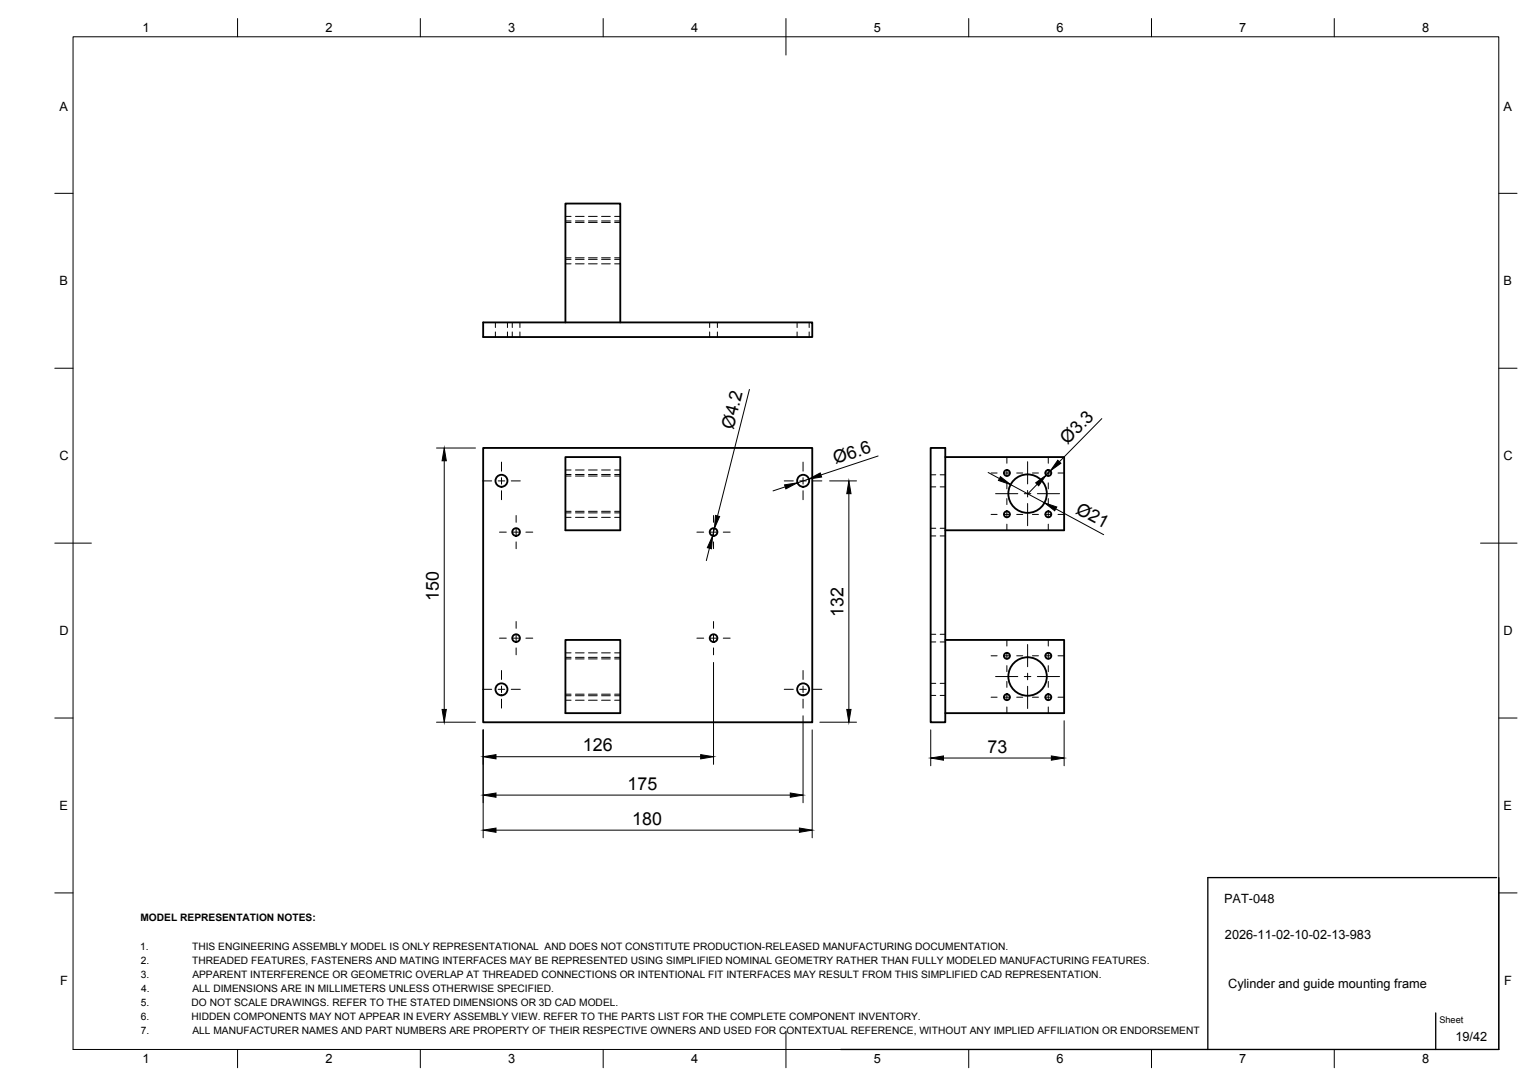
ISO-10303-21;
HEADER;
/* Generated by software containing ST-Developer
 * from STEP Tools, Inc. (www.steptools.com) 
 */

FILE_DESCRIPTION(
/* description */ ('Guided pneumatic stop gate'),
/* implementation_level */ '2;1');

FILE_NAME(
/* name */ 'Cylinder and guide mounting frame.step',
/* time_stamp */ '2026-10-27T21:43:45-07:00',
/* author */ (''),
/* organization */ (''),
/* preprocessor_version */ 'ST-DEVELOPER v20.2',
/* originating_system */ 'Autodesk Translation Framework v15.17.0.0',
/* authorisation */ '');

FILE_SCHEMA (('AUTOMOTIVE_DESIGN { 1 0 10303 214 3 1 1 }'));
ENDSEC;

DATA;
#10=MECHANICAL_DESIGN_GEOMETRIC_PRESENTATION_REPRESENTATION('',(#554),#14392);
#470=SHAPE_REPRESENTATION_RELATIONSHIP('SRR','None',#14605,#512);
#512=ADVANCED_BREP_SHAPE_REPRESENTATION('',(#595),#14367);
#554=STYLED_ITEM('',(#14870),#595);
#595=MANIFOLD_SOLID_BREP('Body1',#7895);
#699=FACE_BOUND('',#1926,.T.);
#700=FACE_BOUND('',#1927,.T.);
#701=FACE_BOUND('',#1928,.T.);
#702=FACE_BOUND('',#1929,.T.);
#703=FACE_BOUND('',#1930,.T.);
#704=FACE_BOUND('',#1932,.T.);
#705=FACE_BOUND('',#1933,.T.);
#706=FACE_BOUND('',#1934,.T.);
#707=FACE_BOUND('',#1935,.T.);
#708=FACE_BOUND('',#1936,.T.);
#709=FACE_BOUND('',#1946,.T.);
#710=FACE_BOUND('',#1947,.T.);
#711=FACE_BOUND('',#1948,.T.);
#712=FACE_BOUND('',#1949,.T.);
#713=FACE_BOUND('',#1950,.T.);
#714=FACE_BOUND('',#1952,.T.);
#715=FACE_BOUND('',#1953,.T.);
#716=FACE_BOUND('',#1954,.T.);
#717=FACE_BOUND('',#1955,.T.);
#718=FACE_BOUND('',#1956,.T.);
#719=FACE_BOUND('',#1962,.T.);
#720=FACE_BOUND('',#1963,.T.);
#721=FACE_BOUND('',#1964,.T.);
#722=FACE_BOUND('',#1965,.T.);
#723=FACE_BOUND('',#1966,.T.);
#724=FACE_BOUND('',#1967,.T.);
#725=FACE_BOUND('',#1968,.T.);
#726=FACE_BOUND('',#1969,.T.);
#727=FACE_BOUND('',#1970,.T.);
#728=FACE_BOUND('',#1971,.T.);
#729=FACE_BOUND('',#1973,.T.);
#730=FACE_BOUND('',#1974,.T.);
#731=FACE_BOUND('',#1975,.T.);
#732=FACE_BOUND('',#1976,.T.);
#733=FACE_BOUND('',#1977,.T.);
#734=FACE_BOUND('',#1978,.T.);
#735=FACE_BOUND('',#1979,.T.);
#736=FACE_BOUND('',#1980,.T.);
#979=PLANE('',#8865);
#980=PLANE('',#8866);
#981=PLANE('',#8867);
#982=PLANE('',#8868);
#983=PLANE('',#8869);
#984=PLANE('',#8885);
#985=PLANE('',#8886);
#986=PLANE('',#8887);
#987=PLANE('',#8888);
#988=PLANE('',#8889);
#989=PLANE('',#8890);
#990=PLANE('',#8891);
#991=PLANE('',#8892);
#992=PLANE('',#8893);
#993=PLANE('',#8894);
#994=PLANE('',#8895);
#1350=FACE_OUTER_BOUND('',#1909,.T.);
#1351=FACE_OUTER_BOUND('',#1910,.T.);
#1352=FACE_OUTER_BOUND('',#1911,.T.);
#1353=FACE_OUTER_BOUND('',#1912,.T.);
#1354=FACE_OUTER_BOUND('',#1913,.T.);
#1355=FACE_OUTER_BOUND('',#1914,.T.);
#1356=FACE_OUTER_BOUND('',#1915,.T.);
#1357=FACE_OUTER_BOUND('',#1916,.T.);
#1358=FACE_OUTER_BOUND('',#1917,.T.);
#1359=FACE_OUTER_BOUND('',#1918,.T.);
#1360=FACE_OUTER_BOUND('',#1919,.T.);
#1361=FACE_OUTER_BOUND('',#1920,.T.);
#1362=FACE_OUTER_BOUND('',#1921,.T.);
#1363=FACE_OUTER_BOUND('',#1922,.T.);
#1364=FACE_OUTER_BOUND('',#1923,.T.);
#1365=FACE_OUTER_BOUND('',#1924,.T.);
#1366=FACE_OUTER_BOUND('',#1925,.T.);
#1367=FACE_OUTER_BOUND('',#1931,.T.);
#1368=FACE_OUTER_BOUND('',#1937,.T.);
#1369=FACE_OUTER_BOUND('',#1938,.T.);
#1370=FACE_OUTER_BOUND('',#1939,.T.);
#1371=FACE_OUTER_BOUND('',#1940,.T.);
#1372=FACE_OUTER_BOUND('',#1941,.T.);
#1373=FACE_OUTER_BOUND('',#1942,.T.);
#1374=FACE_OUTER_BOUND('',#1943,.T.);
#1375=FACE_OUTER_BOUND('',#1944,.T.);
#1376=FACE_OUTER_BOUND('',#1945,.T.);
#1377=FACE_OUTER_BOUND('',#1951,.T.);
#1378=FACE_OUTER_BOUND('',#1957,.T.);
#1379=FACE_OUTER_BOUND('',#1958,.T.);
#1380=FACE_OUTER_BOUND('',#1959,.T.);
#1381=FACE_OUTER_BOUND('',#1960,.T.);
#1382=FACE_OUTER_BOUND('',#1961,.T.);
#1383=FACE_OUTER_BOUND('',#1972,.T.);
#1909=EDGE_LOOP('',(#6222,#6223,#6224,#6225));
#1910=EDGE_LOOP('',(#6226,#6227,#6228,#6229));
#1911=EDGE_LOOP('',(#6230,#6231,#6232,#6233));
#1912=EDGE_LOOP('',(#6234,#6235,#6236,#6237));
#1913=EDGE_LOOP('',(#6238,#6239,#6240,#6241));
#1914=EDGE_LOOP('',(#6242,#6243,#6244,#6245));
#1915=EDGE_LOOP('',(#6246,#6247,#6248,#6249));
#1916=EDGE_LOOP('',(#6250,#6251,#6252,#6253));
#1917=EDGE_LOOP('',(#6254,#6255,#6256,#6257));
#1918=EDGE_LOOP('',(#6258,#6259,#6260,#6261));
#1919=EDGE_LOOP('',(#6262,#6263,#6264,#6265));
#1920=EDGE_LOOP('',(#6266,#6267,#6268,#6269));
#1921=EDGE_LOOP('',(#6270,#6271,#6272,#6273));
#1922=EDGE_LOOP('',(#6274,#6275,#6276,#6277));
#1923=EDGE_LOOP('',(#6278,#6279,#6280,#6281));
#1924=EDGE_LOOP('',(#6282,#6283,#6284,#6285));
#1925=EDGE_LOOP('',(#6286,#6287,#6288,#6289));
#1926=EDGE_LOOP('',(#6290));
#1927=EDGE_LOOP('',(#6291));
#1928=EDGE_LOOP('',(#6292));
#1929=EDGE_LOOP('',(#6293));
#1930=EDGE_LOOP('',(#6294));
#1931=EDGE_LOOP('',(#6295,#6296,#6297,#6298));
#1932=EDGE_LOOP('',(#6299));
#1933=EDGE_LOOP('',(#6300));
#1934=EDGE_LOOP('',(#6301));
#1935=EDGE_LOOP('',(#6302));
#1936=EDGE_LOOP('',(#6303));
#1937=EDGE_LOOP('',(#6304,#6305,#6306,#6307));
#1938=EDGE_LOOP('',(#6308,#6309,#6310,#6311));
#1939=EDGE_LOOP('',(#6312,#6313,#6314,#6315));
#1940=EDGE_LOOP('',(#6316,#6317,#6318,#6319));
#1941=EDGE_LOOP('',(#6320,#6321,#6322,#6323));
#1942=EDGE_LOOP('',(#6324,#6325,#6326,#6327));
#1943=EDGE_LOOP('',(#6328,#6329,#6330,#6331));
#1944=EDGE_LOOP('',(#6332,#6333,#6334,#6335));
#1945=EDGE_LOOP('',(#6336,#6337,#6338,#6339));
#1946=EDGE_LOOP('',(#6340));
#1947=EDGE_LOOP('',(#6341));
#1948=EDGE_LOOP('',(#6342));
#1949=EDGE_LOOP('',(#6343));
#1950=EDGE_LOOP('',(#6344));
#1951=EDGE_LOOP('',(#6345,#6346,#6347,#6348));
#1952=EDGE_LOOP('',(#6349));
#1953=EDGE_LOOP('',(#6350));
#1954=EDGE_LOOP('',(#6351));
#1955=EDGE_LOOP('',(#6352));
#1956=EDGE_LOOP('',(#6353));
#1957=EDGE_LOOP('',(#6354,#6355,#6356,#6357));
#1958=EDGE_LOOP('',(#6358,#6359,#6360,#6361));
#1959=EDGE_LOOP('',(#6362,#6363,#6364,#6365));
#1960=EDGE_LOOP('',(#6366,#6367,#6368,#6369));
#1961=EDGE_LOOP('',(#6370,#6371,#6372,#6373));
#1962=EDGE_LOOP('',(#6374,#6375,#6376,#6377));
#1963=EDGE_LOOP('',(#6378,#6379,#6380,#6381));
#1964=EDGE_LOOP('',(#6382));
#1965=EDGE_LOOP('',(#6383));
#1966=EDGE_LOOP('',(#6384));
#1967=EDGE_LOOP('',(#6385));
#1968=EDGE_LOOP('',(#6386));
#1969=EDGE_LOOP('',(#6387));
#1970=EDGE_LOOP('',(#6388));
#1971=EDGE_LOOP('',(#6389));
#1972=EDGE_LOOP('',(#6390,#6391,#6392,#6393));
#1973=EDGE_LOOP('',(#6394));
#1974=EDGE_LOOP('',(#6395));
#1975=EDGE_LOOP('',(#6396));
#1976=EDGE_LOOP('',(#6397));
#1977=EDGE_LOOP('',(#6398));
#1978=EDGE_LOOP('',(#6399));
#1979=EDGE_LOOP('',(#6400));
#1980=EDGE_LOOP('',(#6401));
#2534=LINE('',#12945,#3079);
#2535=LINE('',#12951,#3080);
#2536=LINE('',#12957,#3081);
#2537=LINE('',#12963,#3082);
#2538=LINE('',#12969,#3083);
#2539=LINE('',#12975,#3084);
#2540=LINE('',#12981,#3085);
#2541=LINE('',#12987,#3086);
#2542=LINE('',#12993,#3087);
#2543=LINE('',#12999,#3088);
#2544=LINE('',#13005,#3089);
#2545=LINE('',#13011,#3090);
#2546=LINE('',#13017,#3091);
#2547=LINE('',#13022,#3092);
#2548=LINE('',#13024,#3093);
#2549=LINE('',#13026,#3094);
#2550=LINE('',#13027,#3095);
#2551=LINE('',#13031,#3096);
#2552=LINE('',#13033,#3097);
#2553=LINE('',#13035,#3098);
#2554=LINE('',#13036,#3099);
#2555=LINE('',#13038,#3100);
#2556=LINE('',#13039,#3101);
#2557=LINE('',#13041,#3102);
#2558=LINE('',#13043,#3103);
#2559=LINE('',#13048,#3104);
#2560=LINE('',#13054,#3105);
#2561=LINE('',#13060,#3106);
#2562=LINE('',#13066,#3107);
#2563=LINE('',#13072,#3108);
#2564=LINE('',#13077,#3109);
#2565=LINE('',#13079,#3110);
#2566=LINE('',#13081,#3111);
#2567=LINE('',#13082,#3112);
#2568=LINE('',#13086,#3113);
#2569=LINE('',#13088,#3114);
#2570=LINE('',#13090,#3115);
#2571=LINE('',#13091,#3116);
#2572=LINE('',#13093,#3117);
#2573=LINE('',#13094,#3118);
#2574=LINE('',#13096,#3119);
#2575=LINE('',#13098,#3120);
#2576=LINE('',#13102,#3121);
#2577=LINE('',#13104,#3122);
#2578=LINE('',#13106,#3123);
#2579=LINE('',#13107,#3124);
#2580=LINE('',#13110,#3125);
#2581=LINE('',#13112,#3126);
#2582=LINE('',#13113,#3127);
#2583=LINE('',#13116,#3128);
#2584=LINE('',#13118,#3129);
#2585=LINE('',#13119,#3130);
#2586=LINE('',#13121,#3131);
#2587=LINE('',#13122,#3132);
#3079=VECTOR('',#10525,0.33);
#3080=VECTOR('',#10532,0.33);
#3081=VECTOR('',#10539,0.33);
#3082=VECTOR('',#10546,0.33);
#3083=VECTOR('',#10553,0.21);
#3084=VECTOR('',#10560,0.21);
#3085=VECTOR('',#10567,0.21);
#3086=VECTOR('',#10574,0.21);
#3087=VECTOR('',#10581,0.165);
#3088=VECTOR('',#10588,0.165);
#3089=VECTOR('',#10595,0.165);
#3090=VECTOR('',#10602,0.165);
#3091=VECTOR('',#10609,1.05);
#3092=VECTOR('',#10614,1.);
#3093=VECTOR('',#10615,1.);
#3094=VECTOR('',#10616,1.);
#3095=VECTOR('',#10617,1.);
#3096=VECTOR('',#10620,1.);
#3097=VECTOR('',#10621,1.);
#3098=VECTOR('',#10622,1.);
#3099=VECTOR('',#10623,1.);
#3100=VECTOR('',#10626,1.);
#3101=VECTOR('',#10627,1.);
#3102=VECTOR('',#10630,1.);
#3103=VECTOR('',#10633,1.);
#3104=VECTOR('',#10638,0.165);
#3105=VECTOR('',#10645,0.165);
#3106=VECTOR('',#10652,0.165);
#3107=VECTOR('',#10659,0.165);
#3108=VECTOR('',#10666,1.05);
#3109=VECTOR('',#10671,1.);
#3110=VECTOR('',#10672,1.);
#3111=VECTOR('',#10673,1.);
#3112=VECTOR('',#10674,1.);
#3113=VECTOR('',#10677,1.);
#3114=VECTOR('',#10678,1.);
#3115=VECTOR('',#10679,1.);
#3116=VECTOR('',#10680,1.);
#3117=VECTOR('',#10683,1.);
#3118=VECTOR('',#10684,1.);
#3119=VECTOR('',#10687,1.);
#3120=VECTOR('',#10690,1.);
#3121=VECTOR('',#10693,1.);
#3122=VECTOR('',#10694,1.);
#3123=VECTOR('',#10695,1.);
#3124=VECTOR('',#10696,1.);
#3125=VECTOR('',#10699,1.);
#3126=VECTOR('',#10700,1.);
#3127=VECTOR('',#10701,1.);
#3128=VECTOR('',#10704,1.);
#3129=VECTOR('',#10705,1.);
#3130=VECTOR('',#10706,1.);
#3131=VECTOR('',#10709,1.);
#3132=VECTOR('',#10710,1.);
#3539=CIRCLE('',#8827,0.33);
#3540=CIRCLE('',#8828,0.33);
#3541=CIRCLE('',#8830,0.33);
#3542=CIRCLE('',#8831,0.33);
#3543=CIRCLE('',#8833,0.33);
#3544=CIRCLE('',#8834,0.33);
#3545=CIRCLE('',#8836,0.33);
#3546=CIRCLE('',#8837,0.33);
#3547=CIRCLE('',#8839,0.21);
#3548=CIRCLE('',#8840,0.21);
#3549=CIRCLE('',#8842,0.21);
#3550=CIRCLE('',#8843,0.21);
#3551=CIRCLE('',#8845,0.21);
#3552=CIRCLE('',#8846,0.21);
#3553=CIRCLE('',#8848,0.21);
#3554=CIRCLE('',#8849,0.21);
#3555=CIRCLE('',#8851,0.165);
#3556=CIRCLE('',#8852,0.165);
#3557=CIRCLE('',#8854,0.165);
#3558=CIRCLE('',#8855,0.165);
#3559=CIRCLE('',#8857,0.165);
#3560=CIRCLE('',#8858,0.165);
#3561=CIRCLE('',#8860,0.165);
#3562=CIRCLE('',#8861,0.165);
#3563=CIRCLE('',#8863,1.05);
#3564=CIRCLE('',#8864,1.05);
#3565=CIRCLE('',#8871,0.165);
#3566=CIRCLE('',#8872,0.165);
#3567=CIRCLE('',#8874,0.165);
#3568=CIRCLE('',#8875,0.165);
#3569=CIRCLE('',#8877,0.165);
#3570=CIRCLE('',#8878,0.165);
#3571=CIRCLE('',#8880,0.165);
#3572=CIRCLE('',#8881,0.165);
#3573=CIRCLE('',#8883,1.05);
#3574=CIRCLE('',#8884,1.05);
#4024=VERTEX_POINT('',#12942);
#4025=VERTEX_POINT('',#12944);
#4026=VERTEX_POINT('',#12948);
#4027=VERTEX_POINT('',#12950);
#4028=VERTEX_POINT('',#12954);
#4029=VERTEX_POINT('',#12956);
#4030=VERTEX_POINT('',#12960);
#4031=VERTEX_POINT('',#12962);
#4032=VERTEX_POINT('',#12966);
#4033=VERTEX_POINT('',#12968);
#4034=VERTEX_POINT('',#12972);
#4035=VERTEX_POINT('',#12974);
#4036=VERTEX_POINT('',#12978);
#4037=VERTEX_POINT('',#12980);
#4038=VERTEX_POINT('',#12984);
#4039=VERTEX_POINT('',#12986);
#4040=VERTEX_POINT('',#12990);
#4041=VERTEX_POINT('',#12992);
#4042=VERTEX_POINT('',#12996);
#4043=VERTEX_POINT('',#12998);
#4044=VERTEX_POINT('',#13002);
#4045=VERTEX_POINT('',#13004);
#4046=VERTEX_POINT('',#13008);
#4047=VERTEX_POINT('',#13010);
#4048=VERTEX_POINT('',#13014);
#4049=VERTEX_POINT('',#13016);
#4050=VERTEX_POINT('',#13020);
#4051=VERTEX_POINT('',#13021);
#4052=VERTEX_POINT('',#13023);
#4053=VERTEX_POINT('',#13025);
#4054=VERTEX_POINT('',#13029);
#4055=VERTEX_POINT('',#13030);
#4056=VERTEX_POINT('',#13032);
#4057=VERTEX_POINT('',#13034);
#4058=VERTEX_POINT('',#13045);
#4059=VERTEX_POINT('',#13047);
#4060=VERTEX_POINT('',#13051);
#4061=VERTEX_POINT('',#13053);
#4062=VERTEX_POINT('',#13057);
#4063=VERTEX_POINT('',#13059);
#4064=VERTEX_POINT('',#13063);
#4065=VERTEX_POINT('',#13065);
#4066=VERTEX_POINT('',#13069);
#4067=VERTEX_POINT('',#13071);
#4068=VERTEX_POINT('',#13075);
#4069=VERTEX_POINT('',#13076);
#4070=VERTEX_POINT('',#13078);
#4071=VERTEX_POINT('',#13080);
#4072=VERTEX_POINT('',#13084);
#4073=VERTEX_POINT('',#13085);
#4074=VERTEX_POINT('',#13087);
#4075=VERTEX_POINT('',#13089);
#4076=VERTEX_POINT('',#13100);
#4077=VERTEX_POINT('',#13101);
#4078=VERTEX_POINT('',#13103);
#4079=VERTEX_POINT('',#13105);
#4080=VERTEX_POINT('',#13109);
#4081=VERTEX_POINT('',#13111);
#4082=VERTEX_POINT('',#13115);
#4083=VERTEX_POINT('',#13117);
#4809=EDGE_CURVE('',#4024,#4024,#3539,.T.);
#4810=EDGE_CURVE('',#4024,#4025,#2534,.T.);
#4811=EDGE_CURVE('',#4025,#4025,#3540,.T.);
#4812=EDGE_CURVE('',#4026,#4026,#3541,.T.);
#4813=EDGE_CURVE('',#4026,#4027,#2535,.T.);
#4814=EDGE_CURVE('',#4027,#4027,#3542,.T.);
#4815=EDGE_CURVE('',#4028,#4028,#3543,.T.);
#4816=EDGE_CURVE('',#4028,#4029,#2536,.T.);
#4817=EDGE_CURVE('',#4029,#4029,#3544,.T.);
#4818=EDGE_CURVE('',#4030,#4030,#3545,.T.);
#4819=EDGE_CURVE('',#4030,#4031,#2537,.T.);
#4820=EDGE_CURVE('',#4031,#4031,#3546,.T.);
#4821=EDGE_CURVE('',#4032,#4032,#3547,.T.);
#4822=EDGE_CURVE('',#4032,#4033,#2538,.T.);
#4823=EDGE_CURVE('',#4033,#4033,#3548,.T.);
#4824=EDGE_CURVE('',#4034,#4034,#3549,.T.);
#4825=EDGE_CURVE('',#4034,#4035,#2539,.T.);
#4826=EDGE_CURVE('',#4035,#4035,#3550,.T.);
#4827=EDGE_CURVE('',#4036,#4036,#3551,.T.);
#4828=EDGE_CURVE('',#4036,#4037,#2540,.T.);
#4829=EDGE_CURVE('',#4037,#4037,#3552,.T.);
#4830=EDGE_CURVE('',#4038,#4038,#3553,.T.);
#4831=EDGE_CURVE('',#4038,#4039,#2541,.T.);
#4832=EDGE_CURVE('',#4039,#4039,#3554,.T.);
#4833=EDGE_CURVE('',#4040,#4040,#3555,.T.);
#4834=EDGE_CURVE('',#4040,#4041,#2542,.T.);
#4835=EDGE_CURVE('',#4041,#4041,#3556,.T.);
#4836=EDGE_CURVE('',#4042,#4042,#3557,.T.);
#4837=EDGE_CURVE('',#4042,#4043,#2543,.T.);
#4838=EDGE_CURVE('',#4043,#4043,#3558,.T.);
#4839=EDGE_CURVE('',#4044,#4044,#3559,.T.);
#4840=EDGE_CURVE('',#4044,#4045,#2544,.T.);
#4841=EDGE_CURVE('',#4045,#4045,#3560,.T.);
#4842=EDGE_CURVE('',#4046,#4046,#3561,.T.);
#4843=EDGE_CURVE('',#4046,#4047,#2545,.T.);
#4844=EDGE_CURVE('',#4047,#4047,#3562,.T.);
#4845=EDGE_CURVE('',#4048,#4048,#3563,.T.);
#4846=EDGE_CURVE('',#4048,#4049,#2546,.T.);
#4847=EDGE_CURVE('',#4049,#4049,#3564,.T.);
#4848=EDGE_CURVE('',#4050,#4051,#2547,.T.);
#4849=EDGE_CURVE('',#4050,#4052,#2548,.T.);
#4850=EDGE_CURVE('',#4053,#4052,#2549,.T.);
#4851=EDGE_CURVE('',#4051,#4053,#2550,.T.);
#4852=EDGE_CURVE('',#4054,#4055,#2551,.T.);
#4853=EDGE_CURVE('',#4056,#4054,#2552,.T.);
#4854=EDGE_CURVE('',#4057,#4056,#2553,.T.);
#4855=EDGE_CURVE('',#4055,#4057,#2554,.T.);
#4856=EDGE_CURVE('',#4055,#4050,#2555,.T.);
#4857=EDGE_CURVE('',#4052,#4057,#2556,.T.);
#4858=EDGE_CURVE('',#4053,#4056,#2557,.T.);
#4859=EDGE_CURVE('',#4054,#4051,#2558,.T.);
#4860=EDGE_CURVE('',#4058,#4058,#3565,.T.);
#4861=EDGE_CURVE('',#4058,#4059,#2559,.T.);
#4862=EDGE_CURVE('',#4059,#4059,#3566,.T.);
#4863=EDGE_CURVE('',#4060,#4060,#3567,.T.);
#4864=EDGE_CURVE('',#4060,#4061,#2560,.T.);
#4865=EDGE_CURVE('',#4061,#4061,#3568,.T.);
#4866=EDGE_CURVE('',#4062,#4062,#3569,.T.);
#4867=EDGE_CURVE('',#4062,#4063,#2561,.T.);
#4868=EDGE_CURVE('',#4063,#4063,#3570,.T.);
#4869=EDGE_CURVE('',#4064,#4064,#3571,.T.);
#4870=EDGE_CURVE('',#4064,#4065,#2562,.T.);
#4871=EDGE_CURVE('',#4065,#4065,#3572,.T.);
#4872=EDGE_CURVE('',#4066,#4066,#3573,.T.);
#4873=EDGE_CURVE('',#4066,#4067,#2563,.T.);
#4874=EDGE_CURVE('',#4067,#4067,#3574,.T.);
#4875=EDGE_CURVE('',#4068,#4069,#2564,.T.);
#4876=EDGE_CURVE('',#4068,#4070,#2565,.T.);
#4877=EDGE_CURVE('',#4071,#4070,#2566,.T.);
#4878=EDGE_CURVE('',#4069,#4071,#2567,.T.);
#4879=EDGE_CURVE('',#4072,#4073,#2568,.T.);
#4880=EDGE_CURVE('',#4074,#4072,#2569,.T.);
#4881=EDGE_CURVE('',#4075,#4074,#2570,.T.);
#4882=EDGE_CURVE('',#4073,#4075,#2571,.T.);
#4883=EDGE_CURVE('',#4073,#4068,#2572,.T.);
#4884=EDGE_CURVE('',#4070,#4075,#2573,.T.);
#4885=EDGE_CURVE('',#4071,#4074,#2574,.T.);
#4886=EDGE_CURVE('',#4072,#4069,#2575,.T.);
#4887=EDGE_CURVE('',#4076,#4077,#2576,.T.);
#4888=EDGE_CURVE('',#4077,#4078,#2577,.T.);
#4889=EDGE_CURVE('',#4079,#4078,#2578,.T.);
#4890=EDGE_CURVE('',#4076,#4079,#2579,.T.);
#4891=EDGE_CURVE('',#4080,#4076,#2580,.T.);
#4892=EDGE_CURVE('',#4081,#4079,#2581,.T.);
#4893=EDGE_CURVE('',#4080,#4081,#2582,.T.);
#4894=EDGE_CURVE('',#4082,#4080,#2583,.T.);
#4895=EDGE_CURVE('',#4083,#4081,#2584,.T.);
#4896=EDGE_CURVE('',#4082,#4083,#2585,.T.);
#4897=EDGE_CURVE('',#4077,#4082,#2586,.T.);
#4898=EDGE_CURVE('',#4078,#4083,#2587,.T.);
#6222=ORIENTED_EDGE('',*,*,#4809,.F.);
#6223=ORIENTED_EDGE('',*,*,#4810,.T.);
#6224=ORIENTED_EDGE('',*,*,#4811,.F.);
#6225=ORIENTED_EDGE('',*,*,#4810,.F.);
#6226=ORIENTED_EDGE('',*,*,#4812,.F.);
#6227=ORIENTED_EDGE('',*,*,#4813,.T.);
#6228=ORIENTED_EDGE('',*,*,#4814,.F.);
#6229=ORIENTED_EDGE('',*,*,#4813,.F.);
#6230=ORIENTED_EDGE('',*,*,#4815,.F.);
#6231=ORIENTED_EDGE('',*,*,#4816,.T.);
#6232=ORIENTED_EDGE('',*,*,#4817,.F.);
#6233=ORIENTED_EDGE('',*,*,#4816,.F.);
#6234=ORIENTED_EDGE('',*,*,#4818,.F.);
#6235=ORIENTED_EDGE('',*,*,#4819,.T.);
#6236=ORIENTED_EDGE('',*,*,#4820,.F.);
#6237=ORIENTED_EDGE('',*,*,#4819,.F.);
#6238=ORIENTED_EDGE('',*,*,#4821,.F.);
#6239=ORIENTED_EDGE('',*,*,#4822,.T.);
#6240=ORIENTED_EDGE('',*,*,#4823,.F.);
#6241=ORIENTED_EDGE('',*,*,#4822,.F.);
#6242=ORIENTED_EDGE('',*,*,#4824,.F.);
#6243=ORIENTED_EDGE('',*,*,#4825,.T.);
#6244=ORIENTED_EDGE('',*,*,#4826,.F.);
#6245=ORIENTED_EDGE('',*,*,#4825,.F.);
#6246=ORIENTED_EDGE('',*,*,#4827,.F.);
#6247=ORIENTED_EDGE('',*,*,#4828,.T.);
#6248=ORIENTED_EDGE('',*,*,#4829,.F.);
#6249=ORIENTED_EDGE('',*,*,#4828,.F.);
#6250=ORIENTED_EDGE('',*,*,#4830,.F.);
#6251=ORIENTED_EDGE('',*,*,#4831,.T.);
#6252=ORIENTED_EDGE('',*,*,#4832,.F.);
#6253=ORIENTED_EDGE('',*,*,#4831,.F.);
#6254=ORIENTED_EDGE('',*,*,#4833,.F.);
#6255=ORIENTED_EDGE('',*,*,#4834,.T.);
#6256=ORIENTED_EDGE('',*,*,#4835,.F.);
#6257=ORIENTED_EDGE('',*,*,#4834,.F.);
#6258=ORIENTED_EDGE('',*,*,#4836,.F.);
#6259=ORIENTED_EDGE('',*,*,#4837,.T.);
#6260=ORIENTED_EDGE('',*,*,#4838,.F.);
#6261=ORIENTED_EDGE('',*,*,#4837,.F.);
#6262=ORIENTED_EDGE('',*,*,#4839,.F.);
#6263=ORIENTED_EDGE('',*,*,#4840,.T.);
#6264=ORIENTED_EDGE('',*,*,#4841,.F.);
#6265=ORIENTED_EDGE('',*,*,#4840,.F.);
#6266=ORIENTED_EDGE('',*,*,#4842,.F.);
#6267=ORIENTED_EDGE('',*,*,#4843,.T.);
#6268=ORIENTED_EDGE('',*,*,#4844,.F.);
#6269=ORIENTED_EDGE('',*,*,#4843,.F.);
#6270=ORIENTED_EDGE('',*,*,#4845,.F.);
#6271=ORIENTED_EDGE('',*,*,#4846,.T.);
#6272=ORIENTED_EDGE('',*,*,#4847,.F.);
#6273=ORIENTED_EDGE('',*,*,#4846,.F.);
#6274=ORIENTED_EDGE('',*,*,#4848,.F.);
#6275=ORIENTED_EDGE('',*,*,#4849,.T.);
#6276=ORIENTED_EDGE('',*,*,#4850,.F.);
#6277=ORIENTED_EDGE('',*,*,#4851,.F.);
#6278=ORIENTED_EDGE('',*,*,#4852,.F.);
#6279=ORIENTED_EDGE('',*,*,#4853,.F.);
#6280=ORIENTED_EDGE('',*,*,#4854,.F.);
#6281=ORIENTED_EDGE('',*,*,#4855,.F.);
#6282=ORIENTED_EDGE('',*,*,#4856,.F.);
#6283=ORIENTED_EDGE('',*,*,#4855,.T.);
#6284=ORIENTED_EDGE('',*,*,#4857,.F.);
#6285=ORIENTED_EDGE('',*,*,#4849,.F.);
#6286=ORIENTED_EDGE('',*,*,#4857,.T.);
#6287=ORIENTED_EDGE('',*,*,#4854,.T.);
#6288=ORIENTED_EDGE('',*,*,#4858,.F.);
#6289=ORIENTED_EDGE('',*,*,#4850,.T.);
#6290=ORIENTED_EDGE('',*,*,#4847,.T.);
#6291=ORIENTED_EDGE('',*,*,#4844,.T.);
#6292=ORIENTED_EDGE('',*,*,#4841,.T.);
#6293=ORIENTED_EDGE('',*,*,#4838,.T.);
#6294=ORIENTED_EDGE('',*,*,#4835,.T.);
#6295=ORIENTED_EDGE('',*,*,#4856,.T.);
#6296=ORIENTED_EDGE('',*,*,#4848,.T.);
#6297=ORIENTED_EDGE('',*,*,#4859,.F.);
#6298=ORIENTED_EDGE('',*,*,#4852,.T.);
#6299=ORIENTED_EDGE('',*,*,#4845,.T.);
#6300=ORIENTED_EDGE('',*,*,#4842,.T.);
#6301=ORIENTED_EDGE('',*,*,#4839,.T.);
#6302=ORIENTED_EDGE('',*,*,#4836,.T.);
#6303=ORIENTED_EDGE('',*,*,#4833,.T.);
#6304=ORIENTED_EDGE('',*,*,#4860,.F.);
#6305=ORIENTED_EDGE('',*,*,#4861,.T.);
#6306=ORIENTED_EDGE('',*,*,#4862,.F.);
#6307=ORIENTED_EDGE('',*,*,#4861,.F.);
#6308=ORIENTED_EDGE('',*,*,#4863,.F.);
#6309=ORIENTED_EDGE('',*,*,#4864,.T.);
#6310=ORIENTED_EDGE('',*,*,#4865,.F.);
#6311=ORIENTED_EDGE('',*,*,#4864,.F.);
#6312=ORIENTED_EDGE('',*,*,#4866,.F.);
#6313=ORIENTED_EDGE('',*,*,#4867,.T.);
#6314=ORIENTED_EDGE('',*,*,#4868,.F.);
#6315=ORIENTED_EDGE('',*,*,#4867,.F.);
#6316=ORIENTED_EDGE('',*,*,#4869,.F.);
#6317=ORIENTED_EDGE('',*,*,#4870,.T.);
#6318=ORIENTED_EDGE('',*,*,#4871,.F.);
#6319=ORIENTED_EDGE('',*,*,#4870,.F.);
#6320=ORIENTED_EDGE('',*,*,#4872,.F.);
#6321=ORIENTED_EDGE('',*,*,#4873,.T.);
#6322=ORIENTED_EDGE('',*,*,#4874,.F.);
#6323=ORIENTED_EDGE('',*,*,#4873,.F.);
#6324=ORIENTED_EDGE('',*,*,#4875,.F.);
#6325=ORIENTED_EDGE('',*,*,#4876,.T.);
#6326=ORIENTED_EDGE('',*,*,#4877,.F.);
#6327=ORIENTED_EDGE('',*,*,#4878,.F.);
#6328=ORIENTED_EDGE('',*,*,#4879,.F.);
#6329=ORIENTED_EDGE('',*,*,#4880,.F.);
#6330=ORIENTED_EDGE('',*,*,#4881,.F.);
#6331=ORIENTED_EDGE('',*,*,#4882,.F.);
#6332=ORIENTED_EDGE('',*,*,#4883,.F.);
#6333=ORIENTED_EDGE('',*,*,#4882,.T.);
#6334=ORIENTED_EDGE('',*,*,#4884,.F.);
#6335=ORIENTED_EDGE('',*,*,#4876,.F.);
#6336=ORIENTED_EDGE('',*,*,#4884,.T.);
#6337=ORIENTED_EDGE('',*,*,#4881,.T.);
#6338=ORIENTED_EDGE('',*,*,#4885,.F.);
#6339=ORIENTED_EDGE('',*,*,#4877,.T.);
#6340=ORIENTED_EDGE('',*,*,#4874,.T.);
#6341=ORIENTED_EDGE('',*,*,#4871,.T.);
#6342=ORIENTED_EDGE('',*,*,#4868,.T.);
#6343=ORIENTED_EDGE('',*,*,#4865,.T.);
#6344=ORIENTED_EDGE('',*,*,#4862,.T.);
#6345=ORIENTED_EDGE('',*,*,#4883,.T.);
#6346=ORIENTED_EDGE('',*,*,#4875,.T.);
#6347=ORIENTED_EDGE('',*,*,#4886,.F.);
#6348=ORIENTED_EDGE('',*,*,#4879,.T.);
#6349=ORIENTED_EDGE('',*,*,#4872,.T.);
#6350=ORIENTED_EDGE('',*,*,#4869,.T.);
#6351=ORIENTED_EDGE('',*,*,#4866,.T.);
#6352=ORIENTED_EDGE('',*,*,#4863,.T.);
#6353=ORIENTED_EDGE('',*,*,#4860,.T.);
#6354=ORIENTED_EDGE('',*,*,#4887,.T.);
#6355=ORIENTED_EDGE('',*,*,#4888,.T.);
#6356=ORIENTED_EDGE('',*,*,#4889,.F.);
#6357=ORIENTED_EDGE('',*,*,#4890,.F.);
#6358=ORIENTED_EDGE('',*,*,#4891,.T.);
#6359=ORIENTED_EDGE('',*,*,#4890,.T.);
#6360=ORIENTED_EDGE('',*,*,#4892,.F.);
#6361=ORIENTED_EDGE('',*,*,#4893,.F.);
#6362=ORIENTED_EDGE('',*,*,#4894,.T.);
#6363=ORIENTED_EDGE('',*,*,#4893,.T.);
#6364=ORIENTED_EDGE('',*,*,#4895,.F.);
#6365=ORIENTED_EDGE('',*,*,#4896,.F.);
#6366=ORIENTED_EDGE('',*,*,#4897,.T.);
#6367=ORIENTED_EDGE('',*,*,#4896,.T.);
#6368=ORIENTED_EDGE('',*,*,#4898,.F.);
#6369=ORIENTED_EDGE('',*,*,#4888,.F.);
#6370=ORIENTED_EDGE('',*,*,#4898,.T.);
#6371=ORIENTED_EDGE('',*,*,#4895,.T.);
#6372=ORIENTED_EDGE('',*,*,#4892,.T.);
#6373=ORIENTED_EDGE('',*,*,#4889,.T.);
#6374=ORIENTED_EDGE('',*,*,#4880,.T.);
#6375=ORIENTED_EDGE('',*,*,#4886,.T.);
#6376=ORIENTED_EDGE('',*,*,#4878,.T.);
#6377=ORIENTED_EDGE('',*,*,#4885,.T.);
#6378=ORIENTED_EDGE('',*,*,#4853,.T.);
#6379=ORIENTED_EDGE('',*,*,#4859,.T.);
#6380=ORIENTED_EDGE('',*,*,#4851,.T.);
#6381=ORIENTED_EDGE('',*,*,#4858,.T.);
#6382=ORIENTED_EDGE('',*,*,#4832,.T.);
#6383=ORIENTED_EDGE('',*,*,#4829,.T.);
#6384=ORIENTED_EDGE('',*,*,#4826,.T.);
#6385=ORIENTED_EDGE('',*,*,#4823,.T.);
#6386=ORIENTED_EDGE('',*,*,#4820,.T.);
#6387=ORIENTED_EDGE('',*,*,#4817,.T.);
#6388=ORIENTED_EDGE('',*,*,#4814,.T.);
#6389=ORIENTED_EDGE('',*,*,#4811,.T.);
#6390=ORIENTED_EDGE('',*,*,#4897,.F.);
#6391=ORIENTED_EDGE('',*,*,#4887,.F.);
#6392=ORIENTED_EDGE('',*,*,#4891,.F.);
#6393=ORIENTED_EDGE('',*,*,#4894,.F.);
#6394=ORIENTED_EDGE('',*,*,#4830,.T.);
#6395=ORIENTED_EDGE('',*,*,#4827,.T.);
#6396=ORIENTED_EDGE('',*,*,#4824,.T.);
#6397=ORIENTED_EDGE('',*,*,#4821,.T.);
#6398=ORIENTED_EDGE('',*,*,#4818,.T.);
#6399=ORIENTED_EDGE('',*,*,#4815,.T.);
#6400=ORIENTED_EDGE('',*,*,#4812,.T.);
#6401=ORIENTED_EDGE('',*,*,#4809,.T.);
#7315=CYLINDRICAL_SURFACE('',#8826,0.33);
#7316=CYLINDRICAL_SURFACE('',#8829,0.33);
#7317=CYLINDRICAL_SURFACE('',#8832,0.33);
#7318=CYLINDRICAL_SURFACE('',#8835,0.33);
#7319=CYLINDRICAL_SURFACE('',#8838,0.21);
#7320=CYLINDRICAL_SURFACE('',#8841,0.21);
#7321=CYLINDRICAL_SURFACE('',#8844,0.21);
#7322=CYLINDRICAL_SURFACE('',#8847,0.21);
#7323=CYLINDRICAL_SURFACE('',#8850,0.165);
#7324=CYLINDRICAL_SURFACE('',#8853,0.165);
#7325=CYLINDRICAL_SURFACE('',#8856,0.165);
#7326=CYLINDRICAL_SURFACE('',#8859,0.165);
#7327=CYLINDRICAL_SURFACE('',#8862,1.05);
#7328=CYLINDRICAL_SURFACE('',#8870,0.165);
#7329=CYLINDRICAL_SURFACE('',#8873,0.165);
#7330=CYLINDRICAL_SURFACE('',#8876,0.165);
#7331=CYLINDRICAL_SURFACE('',#8879,0.165);
#7332=CYLINDRICAL_SURFACE('',#8882,1.05);
#7632=ADVANCED_FACE('',(#1350),#7315,.F.);
#7633=ADVANCED_FACE('',(#1351),#7316,.F.);
#7634=ADVANCED_FACE('',(#1352),#7317,.F.);
#7635=ADVANCED_FACE('',(#1353),#7318,.F.);
#7636=ADVANCED_FACE('',(#1354),#7319,.F.);
#7637=ADVANCED_FACE('',(#1355),#7320,.F.);
#7638=ADVANCED_FACE('',(#1356),#7321,.F.);
#7639=ADVANCED_FACE('',(#1357),#7322,.F.);
#7640=ADVANCED_FACE('',(#1358),#7323,.F.);
#7641=ADVANCED_FACE('',(#1359),#7324,.F.);
#7642=ADVANCED_FACE('',(#1360),#7325,.F.);
#7643=ADVANCED_FACE('',(#1361),#7326,.F.);
#7644=ADVANCED_FACE('',(#1362),#7327,.F.);
#7645=ADVANCED_FACE('',(#1363),#979,.T.);
#7646=ADVANCED_FACE('',(#1364),#980,.T.);
#7647=ADVANCED_FACE('',(#1365),#981,.T.);
#7648=ADVANCED_FACE('',(#1366,#699,#700,#701,#702,#703),#982,.T.);
#7649=ADVANCED_FACE('',(#1367,#704,#705,#706,#707,#708),#983,.F.);
#7650=ADVANCED_FACE('',(#1368),#7328,.F.);
#7651=ADVANCED_FACE('',(#1369),#7329,.F.);
#7652=ADVANCED_FACE('',(#1370),#7330,.F.);
#7653=ADVANCED_FACE('',(#1371),#7331,.F.);
#7654=ADVANCED_FACE('',(#1372),#7332,.F.);
#7655=ADVANCED_FACE('',(#1373),#984,.T.);
#7656=ADVANCED_FACE('',(#1374),#985,.T.);
#7657=ADVANCED_FACE('',(#1375),#986,.T.);
#7658=ADVANCED_FACE('',(#1376,#709,#710,#711,#712,#713),#987,.T.);
#7659=ADVANCED_FACE('',(#1377,#714,#715,#716,#717,#718),#988,.F.);
#7660=ADVANCED_FACE('',(#1378),#989,.T.);
#7661=ADVANCED_FACE('',(#1379),#990,.T.);
#7662=ADVANCED_FACE('',(#1380),#991,.T.);
#7663=ADVANCED_FACE('',(#1381),#992,.T.);
#7664=ADVANCED_FACE('',(#1382,#719,#720,#721,#722,#723,#724,#725,#726,#727,
#728),#993,.T.);
#7665=ADVANCED_FACE('',(#1383,#729,#730,#731,#732,#733,#734,#735,#736),
#994,.F.);
#7895=CLOSED_SHELL('',(#7632,#7633,#7634,#7635,#7636,#7637,#7638,#7639,
#7640,#7641,#7642,#7643,#7644,#7645,#7646,#7647,#7648,#7649,#7650,#7651,
#7652,#7653,#7654,#7655,#7656,#7657,#7658,#7659,#7660,#7661,#7662,#7663,
#7664,#7665));
#8825=AXIS2_PLACEMENT_3D('',#12940,#10519,#10520);
#8826=AXIS2_PLACEMENT_3D('',#12941,#10521,#10522);
#8827=AXIS2_PLACEMENT_3D('',#12943,#10523,#10524);
#8828=AXIS2_PLACEMENT_3D('',#12946,#10526,#10527);
#8829=AXIS2_PLACEMENT_3D('',#12947,#10528,#10529);
#8830=AXIS2_PLACEMENT_3D('',#12949,#10530,#10531);
#8831=AXIS2_PLACEMENT_3D('',#12952,#10533,#10534);
#8832=AXIS2_PLACEMENT_3D('',#12953,#10535,#10536);
#8833=AXIS2_PLACEMENT_3D('',#12955,#10537,#10538);
#8834=AXIS2_PLACEMENT_3D('',#12958,#10540,#10541);
#8835=AXIS2_PLACEMENT_3D('',#12959,#10542,#10543);
#8836=AXIS2_PLACEMENT_3D('',#12961,#10544,#10545);
#8837=AXIS2_PLACEMENT_3D('',#12964,#10547,#10548);
#8838=AXIS2_PLACEMENT_3D('',#12965,#10549,#10550);
#8839=AXIS2_PLACEMENT_3D('',#12967,#10551,#10552);
#8840=AXIS2_PLACEMENT_3D('',#12970,#10554,#10555);
#8841=AXIS2_PLACEMENT_3D('',#12971,#10556,#10557);
#8842=AXIS2_PLACEMENT_3D('',#12973,#10558,#10559);
#8843=AXIS2_PLACEMENT_3D('',#12976,#10561,#10562);
#8844=AXIS2_PLACEMENT_3D('',#12977,#10563,#10564);
#8845=AXIS2_PLACEMENT_3D('',#12979,#10565,#10566);
#8846=AXIS2_PLACEMENT_3D('',#12982,#10568,#10569);
#8847=AXIS2_PLACEMENT_3D('',#12983,#10570,#10571);
#8848=AXIS2_PLACEMENT_3D('',#12985,#10572,#10573);
#8849=AXIS2_PLACEMENT_3D('',#12988,#10575,#10576);
#8850=AXIS2_PLACEMENT_3D('',#12989,#10577,#10578);
#8851=AXIS2_PLACEMENT_3D('',#12991,#10579,#10580);
#8852=AXIS2_PLACEMENT_3D('',#12994,#10582,#10583);
#8853=AXIS2_PLACEMENT_3D('',#12995,#10584,#10585);
#8854=AXIS2_PLACEMENT_3D('',#12997,#10586,#10587);
#8855=AXIS2_PLACEMENT_3D('',#13000,#10589,#10590);
#8856=AXIS2_PLACEMENT_3D('',#13001,#10591,#10592);
#8857=AXIS2_PLACEMENT_3D('',#13003,#10593,#10594);
#8858=AXIS2_PLACEMENT_3D('',#13006,#10596,#10597);
#8859=AXIS2_PLACEMENT_3D('',#13007,#10598,#10599);
#8860=AXIS2_PLACEMENT_3D('',#13009,#10600,#10601);
#8861=AXIS2_PLACEMENT_3D('',#13012,#10603,#10604);
#8862=AXIS2_PLACEMENT_3D('',#13013,#10605,#10606);
#8863=AXIS2_PLACEMENT_3D('',#13015,#10607,#10608);
#8864=AXIS2_PLACEMENT_3D('',#13018,#10610,#10611);
#8865=AXIS2_PLACEMENT_3D('',#13019,#10612,#10613);
#8866=AXIS2_PLACEMENT_3D('',#13028,#10618,#10619);
#8867=AXIS2_PLACEMENT_3D('',#13037,#10624,#10625);
#8868=AXIS2_PLACEMENT_3D('',#13040,#10628,#10629);
#8869=AXIS2_PLACEMENT_3D('',#13042,#10631,#10632);
#8870=AXIS2_PLACEMENT_3D('',#13044,#10634,#10635);
#8871=AXIS2_PLACEMENT_3D('',#13046,#10636,#10637);
#8872=AXIS2_PLACEMENT_3D('',#13049,#10639,#10640);
#8873=AXIS2_PLACEMENT_3D('',#13050,#10641,#10642);
#8874=AXIS2_PLACEMENT_3D('',#13052,#10643,#10644);
#8875=AXIS2_PLACEMENT_3D('',#13055,#10646,#10647);
#8876=AXIS2_PLACEMENT_3D('',#13056,#10648,#10649);
#8877=AXIS2_PLACEMENT_3D('',#13058,#10650,#10651);
#8878=AXIS2_PLACEMENT_3D('',#13061,#10653,#10654);
#8879=AXIS2_PLACEMENT_3D('',#13062,#10655,#10656);
#8880=AXIS2_PLACEMENT_3D('',#13064,#10657,#10658);
#8881=AXIS2_PLACEMENT_3D('',#13067,#10660,#10661);
#8882=AXIS2_PLACEMENT_3D('',#13068,#10662,#10663);
#8883=AXIS2_PLACEMENT_3D('',#13070,#10664,#10665);
#8884=AXIS2_PLACEMENT_3D('',#13073,#10667,#10668);
#8885=AXIS2_PLACEMENT_3D('',#13074,#10669,#10670);
#8886=AXIS2_PLACEMENT_3D('',#13083,#10675,#10676);
#8887=AXIS2_PLACEMENT_3D('',#13092,#10681,#10682);
#8888=AXIS2_PLACEMENT_3D('',#13095,#10685,#10686);
#8889=AXIS2_PLACEMENT_3D('',#13097,#10688,#10689);
#8890=AXIS2_PLACEMENT_3D('',#13099,#10691,#10692);
#8891=AXIS2_PLACEMENT_3D('',#13108,#10697,#10698);
#8892=AXIS2_PLACEMENT_3D('',#13114,#10702,#10703);
#8893=AXIS2_PLACEMENT_3D('',#13120,#10707,#10708);
#8894=AXIS2_PLACEMENT_3D('',#13123,#10711,#10712);
#8895=AXIS2_PLACEMENT_3D('',#13124,#10713,#10714);
#10519=DIRECTION('axis',(0.,0.,1.));
#10520=DIRECTION('refdir',(1.,0.,0.));
#10521=DIRECTION('center_axis',(0.,0.,1.));
#10522=DIRECTION('ref_axis',(1.,0.,0.));
#10523=DIRECTION('center_axis',(0.,0.,1.));
#10524=DIRECTION('ref_axis',(1.,0.,0.));
#10525=DIRECTION('',(0.,0.,1.));
#10526=DIRECTION('center_axis',(0.,0.,-1.));
#10527=DIRECTION('ref_axis',(1.,0.,0.));
#10528=DIRECTION('center_axis',(0.,0.,1.));
#10529=DIRECTION('ref_axis',(1.,0.,0.));
#10530=DIRECTION('center_axis',(0.,0.,1.));
#10531=DIRECTION('ref_axis',(1.,0.,0.));
#10532=DIRECTION('',(0.,0.,1.));
#10533=DIRECTION('center_axis',(0.,0.,-1.));
#10534=DIRECTION('ref_axis',(1.,0.,0.));
#10535=DIRECTION('center_axis',(0.,0.,1.));
#10536=DIRECTION('ref_axis',(1.,0.,0.));
#10537=DIRECTION('center_axis',(0.,0.,1.));
#10538=DIRECTION('ref_axis',(1.,0.,0.));
#10539=DIRECTION('',(0.,0.,1.));
#10540=DIRECTION('center_axis',(0.,0.,-1.));
#10541=DIRECTION('ref_axis',(1.,0.,0.));
#10542=DIRECTION('center_axis',(0.,0.,1.));
#10543=DIRECTION('ref_axis',(1.,0.,0.));
#10544=DIRECTION('center_axis',(0.,0.,1.));
#10545=DIRECTION('ref_axis',(1.,0.,0.));
#10546=DIRECTION('',(0.,0.,1.));
#10547=DIRECTION('center_axis',(0.,0.,-1.));
#10548=DIRECTION('ref_axis',(1.,0.,0.));
#10549=DIRECTION('center_axis',(0.,0.,1.));
#10550=DIRECTION('ref_axis',(1.,0.,0.));
#10551=DIRECTION('center_axis',(0.,0.,1.));
#10552=DIRECTION('ref_axis',(1.,0.,0.));
#10553=DIRECTION('',(0.,0.,1.));
#10554=DIRECTION('center_axis',(0.,0.,-1.));
#10555=DIRECTION('ref_axis',(1.,0.,0.));
#10556=DIRECTION('center_axis',(0.,0.,1.));
#10557=DIRECTION('ref_axis',(1.,0.,0.));
#10558=DIRECTION('center_axis',(0.,0.,1.));
#10559=DIRECTION('ref_axis',(1.,0.,0.));
#10560=DIRECTION('',(0.,0.,1.));
#10561=DIRECTION('center_axis',(0.,0.,-1.));
#10562=DIRECTION('ref_axis',(1.,0.,0.));
#10563=DIRECTION('center_axis',(0.,0.,1.));
#10564=DIRECTION('ref_axis',(1.,0.,0.));
#10565=DIRECTION('center_axis',(0.,0.,1.));
#10566=DIRECTION('ref_axis',(1.,0.,0.));
#10567=DIRECTION('',(0.,0.,1.));
#10568=DIRECTION('center_axis',(0.,0.,-1.));
#10569=DIRECTION('ref_axis',(1.,0.,0.));
#10570=DIRECTION('center_axis',(0.,0.,1.));
#10571=DIRECTION('ref_axis',(1.,0.,0.));
#10572=DIRECTION('center_axis',(0.,0.,1.));
#10573=DIRECTION('ref_axis',(1.,0.,0.));
#10574=DIRECTION('',(0.,0.,1.));
#10575=DIRECTION('center_axis',(0.,0.,-1.));
#10576=DIRECTION('ref_axis',(1.,0.,0.));
#10577=DIRECTION('center_axis',(0.,1.,0.));
#10578=DIRECTION('ref_axis',(1.,0.,0.));
#10579=DIRECTION('center_axis',(0.,1.,0.));
#10580=DIRECTION('ref_axis',(1.,0.,0.));
#10581=DIRECTION('',(0.,1.,0.));
#10582=DIRECTION('center_axis',(0.,-1.,0.));
#10583=DIRECTION('ref_axis',(1.,0.,0.));
#10584=DIRECTION('center_axis',(0.,1.,0.));
#10585=DIRECTION('ref_axis',(1.,0.,0.));
#10586=DIRECTION('center_axis',(0.,1.,0.));
#10587=DIRECTION('ref_axis',(1.,0.,0.));
#10588=DIRECTION('',(0.,1.,0.));
#10589=DIRECTION('center_axis',(0.,-1.,0.));
#10590=DIRECTION('ref_axis',(1.,0.,0.));
#10591=DIRECTION('center_axis',(0.,1.,0.));
#10592=DIRECTION('ref_axis',(1.,0.,0.));
#10593=DIRECTION('center_axis',(0.,1.,0.));
#10594=DIRECTION('ref_axis',(1.,0.,0.));
#10595=DIRECTION('',(0.,1.,0.));
#10596=DIRECTION('center_axis',(0.,-1.,0.));
#10597=DIRECTION('ref_axis',(1.,0.,0.));
#10598=DIRECTION('center_axis',(0.,1.,0.));
#10599=DIRECTION('ref_axis',(1.,0.,0.));
#10600=DIRECTION('center_axis',(0.,1.,0.));
#10601=DIRECTION('ref_axis',(1.,0.,0.));
#10602=DIRECTION('',(0.,1.,0.));
#10603=DIRECTION('center_axis',(0.,-1.,0.));
#10604=DIRECTION('ref_axis',(1.,0.,0.));
#10605=DIRECTION('center_axis',(0.,1.,0.));
#10606=DIRECTION('ref_axis',(1.,0.,0.));
#10607=DIRECTION('center_axis',(0.,1.,0.));
#10608=DIRECTION('ref_axis',(1.,0.,0.));
#10609=DIRECTION('',(0.,1.,0.));
#10610=DIRECTION('center_axis',(0.,-1.,0.));
#10611=DIRECTION('ref_axis',(1.,0.,0.));
#10612=DIRECTION('center_axis',(-1.,0.,0.));
#10613=DIRECTION('ref_axis',(0.,0.,1.));
#10614=DIRECTION('',(0.,0.,-1.));
#10615=DIRECTION('',(0.,1.,0.));
#10616=DIRECTION('',(0.,0.,1.));
#10617=DIRECTION('',(0.,1.,0.));
#10618=DIRECTION('center_axis',(1.,0.,0.));
#10619=DIRECTION('ref_axis',(0.,0.,-1.));
#10620=DIRECTION('',(0.,0.,1.));
#10621=DIRECTION('',(0.,-1.,0.));
#10622=DIRECTION('',(0.,0.,-1.));
#10623=DIRECTION('',(0.,1.,0.));
#10624=DIRECTION('center_axis',(0.,0.,1.));
#10625=DIRECTION('ref_axis',(1.,0.,0.));
#10626=DIRECTION('',(-1.,0.,0.));
#10627=DIRECTION('',(1.,0.,0.));
#10628=DIRECTION('center_axis',(0.,1.,0.));
#10629=DIRECTION('ref_axis',(0.,0.,1.));
#10630=DIRECTION('',(1.,0.,0.));
#10631=DIRECTION('center_axis',(0.,1.,0.));
#10632=DIRECTION('ref_axis',(1.,0.,0.));
#10633=DIRECTION('',(-1.,0.,0.));
#10634=DIRECTION('center_axis',(0.,1.,0.));
#10635=DIRECTION('ref_axis',(1.,0.,0.));
#10636=DIRECTION('center_axis',(0.,1.,0.));
#10637=DIRECTION('ref_axis',(1.,0.,0.));
#10638=DIRECTION('',(0.,1.,0.));
#10639=DIRECTION('center_axis',(0.,-1.,0.));
#10640=DIRECTION('ref_axis',(1.,0.,0.));
#10641=DIRECTION('center_axis',(0.,1.,0.));
#10642=DIRECTION('ref_axis',(1.,0.,0.));
#10643=DIRECTION('center_axis',(0.,1.,0.));
#10644=DIRECTION('ref_axis',(1.,0.,0.));
#10645=DIRECTION('',(0.,1.,0.));
#10646=DIRECTION('center_axis',(0.,-1.,0.));
#10647=DIRECTION('ref_axis',(1.,0.,0.));
#10648=DIRECTION('center_axis',(0.,1.,0.));
#10649=DIRECTION('ref_axis',(1.,0.,0.));
#10650=DIRECTION('center_axis',(0.,1.,0.));
#10651=DIRECTION('ref_axis',(1.,0.,0.));
#10652=DIRECTION('',(0.,1.,0.));
#10653=DIRECTION('center_axis',(0.,-1.,0.));
#10654=DIRECTION('ref_axis',(1.,0.,0.));
#10655=DIRECTION('center_axis',(0.,1.,0.));
#10656=DIRECTION('ref_axis',(1.,0.,0.));
#10657=DIRECTION('center_axis',(0.,1.,0.));
#10658=DIRECTION('ref_axis',(1.,0.,0.));
#10659=DIRECTION('',(0.,1.,0.));
#10660=DIRECTION('center_axis',(0.,-1.,0.));
#10661=DIRECTION('ref_axis',(1.,0.,0.));
#10662=DIRECTION('center_axis',(0.,1.,0.));
#10663=DIRECTION('ref_axis',(1.,0.,0.));
#10664=DIRECTION('center_axis',(0.,1.,0.));
#10665=DIRECTION('ref_axis',(1.,0.,0.));
#10666=DIRECTION('',(0.,1.,0.));
#10667=DIRECTION('center_axis',(0.,-1.,0.));
#10668=DIRECTION('ref_axis',(1.,0.,0.));
#10669=DIRECTION('center_axis',(-1.,0.,0.));
#10670=DIRECTION('ref_axis',(0.,0.,1.));
#10671=DIRECTION('',(0.,0.,-1.));
#10672=DIRECTION('',(0.,1.,0.));
#10673=DIRECTION('',(0.,0.,1.));
#10674=DIRECTION('',(0.,1.,0.));
#10675=DIRECTION('center_axis',(1.,0.,0.));
#10676=DIRECTION('ref_axis',(0.,0.,-1.));
#10677=DIRECTION('',(0.,0.,1.));
#10678=DIRECTION('',(0.,-1.,0.));
#10679=DIRECTION('',(0.,0.,-1.));
#10680=DIRECTION('',(0.,1.,0.));
#10681=DIRECTION('center_axis',(0.,0.,1.));
#10682=DIRECTION('ref_axis',(1.,0.,0.));
#10683=DIRECTION('',(-1.,0.,0.));
#10684=DIRECTION('',(1.,0.,0.));
#10685=DIRECTION('center_axis',(0.,1.,0.));
#10686=DIRECTION('ref_axis',(0.,0.,1.));
#10687=DIRECTION('',(1.,0.,0.));
#10688=DIRECTION('center_axis',(0.,1.,0.));
#10689=DIRECTION('ref_axis',(1.,0.,0.));
#10690=DIRECTION('',(-1.,0.,0.));
#10691=DIRECTION('center_axis',(0.,1.,0.));
#10692=DIRECTION('ref_axis',(-1.,0.,0.));
#10693=DIRECTION('',(-1.,0.,0.));
#10694=DIRECTION('',(0.,0.,1.));
#10695=DIRECTION('',(-1.,0.,0.));
#10696=DIRECTION('',(0.,0.,1.));
#10697=DIRECTION('center_axis',(1.,0.,0.));
#10698=DIRECTION('ref_axis',(0.,1.,0.));
#10699=DIRECTION('',(0.,1.,0.));
#10700=DIRECTION('',(0.,1.,0.));
#10701=DIRECTION('',(0.,0.,1.));
#10702=DIRECTION('center_axis',(0.,-1.,0.));
#10703=DIRECTION('ref_axis',(1.,0.,0.));
#10704=DIRECTION('',(1.,0.,0.));
#10705=DIRECTION('',(1.,0.,0.));
#10706=DIRECTION('',(0.,0.,1.));
#10707=DIRECTION('center_axis',(-1.,0.,0.));
#10708=DIRECTION('ref_axis',(0.,-1.,0.));
#10709=DIRECTION('',(0.,-1.,0.));
#10710=DIRECTION('',(0.,-1.,0.));
#10711=DIRECTION('center_axis',(0.,0.,1.));
#10712=DIRECTION('ref_axis',(1.,0.,0.));
#10713=DIRECTION('center_axis',(0.,0.,1.));
#10714=DIRECTION('ref_axis',(1.,0.,0.));
#12940=CARTESIAN_POINT('',(0.,0.,0.));
#12941=CARTESIAN_POINT('Origin',(5.7,-4.,-0.9));
#12942=CARTESIAN_POINT('',(5.37,-4.,-0.8));
#12943=CARTESIAN_POINT('Origin',(5.7,-4.,-0.8));
#12944=CARTESIAN_POINT('',(5.37,-4.,0.));
#12945=CARTESIAN_POINT('',(5.37,-4.,-0.9));
#12946=CARTESIAN_POINT('Origin',(5.7,-4.,0.));
#12947=CARTESIAN_POINT('Origin',(-5.7,12.5,-0.9));
#12948=CARTESIAN_POINT('',(-6.03,12.5,-0.8));
#12949=CARTESIAN_POINT('Origin',(-5.7,12.5,-0.8));
#12950=CARTESIAN_POINT('',(-6.03,12.5,0.));
#12951=CARTESIAN_POINT('',(-6.03,12.5,-0.9));
#12952=CARTESIAN_POINT('Origin',(-5.7,12.5,0.));
#12953=CARTESIAN_POINT('Origin',(-5.7,-4.,-0.9));
#12954=CARTESIAN_POINT('',(-6.03,-4.,-0.8));
#12955=CARTESIAN_POINT('Origin',(-5.7,-4.,-0.8));
#12956=CARTESIAN_POINT('',(-6.03,-4.,0.));
#12957=CARTESIAN_POINT('',(-6.03,-4.,-0.9));
#12958=CARTESIAN_POINT('Origin',(-5.7,-4.,0.));
#12959=CARTESIAN_POINT('Origin',(5.7,12.5,-0.9));
#12960=CARTESIAN_POINT('',(5.37,12.5,-0.8));
#12961=CARTESIAN_POINT('Origin',(5.7,12.5,-0.8));
#12962=CARTESIAN_POINT('',(5.37,12.5,0.));
#12963=CARTESIAN_POINT('',(5.37,12.5,-0.9));
#12964=CARTESIAN_POINT('Origin',(5.7,12.5,0.));
#12965=CARTESIAN_POINT('Origin',(2.9,11.7,-0.9));
#12966=CARTESIAN_POINT('',(2.69,11.7,-0.8));
#12967=CARTESIAN_POINT('Origin',(2.9,11.7,-0.8));
#12968=CARTESIAN_POINT('',(2.69,11.7,0.));
#12969=CARTESIAN_POINT('',(2.69,11.7,-0.9));
#12970=CARTESIAN_POINT('Origin',(2.9,11.7,0.));
#12971=CARTESIAN_POINT('Origin',(2.9,0.9,-0.9));
#12972=CARTESIAN_POINT('',(2.69,0.9,-0.8));
#12973=CARTESIAN_POINT('Origin',(2.9,0.9,-0.8));
#12974=CARTESIAN_POINT('',(2.69,0.9,0.));
#12975=CARTESIAN_POINT('',(2.69,0.9,-0.9));
#12976=CARTESIAN_POINT('Origin',(2.9,0.9,0.));
#12977=CARTESIAN_POINT('Origin',(-2.9,11.7,-0.9));
#12978=CARTESIAN_POINT('',(-3.11,11.7,-0.8));
#12979=CARTESIAN_POINT('Origin',(-2.9,11.7,-0.8));
#12980=CARTESIAN_POINT('',(-3.11,11.7,0.));
#12981=CARTESIAN_POINT('',(-3.11,11.7,-0.9));
#12982=CARTESIAN_POINT('Origin',(-2.9,11.7,0.));
#12983=CARTESIAN_POINT('Origin',(-2.9,0.9,-0.9));
#12984=CARTESIAN_POINT('',(-3.11,0.9,-0.8));
#12985=CARTESIAN_POINT('Origin',(-2.9,0.9,-0.8));
#12986=CARTESIAN_POINT('',(-3.11,0.9,0.));
#12987=CARTESIAN_POINT('',(-3.11,0.9,-0.9));
#12988=CARTESIAN_POINT('Origin',(-2.9,0.9,0.));
#12989=CARTESIAN_POINT('Origin',(3.86862915010152,5.9,3.36862915010152));
#12990=CARTESIAN_POINT('',(3.70362915010152,6.,3.36862915010152));
#12991=CARTESIAN_POINT('Origin',(3.86862915010152,6.,3.36862915010152));
#12992=CARTESIAN_POINT('',(3.70362915010152,9.,3.36862915010152));
#12993=CARTESIAN_POINT('',(3.70362915010152,5.9,3.36862915010152));
#12994=CARTESIAN_POINT('Origin',(3.86862915010152,9.,3.36862915010152));
#12995=CARTESIAN_POINT('Origin',(3.86862915010152,5.9,5.63137084989848));
#12996=CARTESIAN_POINT('',(3.70362915010152,6.,5.63137084989848));
#12997=CARTESIAN_POINT('Origin',(3.86862915010152,6.,5.63137084989848));
#12998=CARTESIAN_POINT('',(3.70362915010152,9.,5.63137084989848));
#12999=CARTESIAN_POINT('',(3.70362915010152,5.9,5.63137084989848));
#13000=CARTESIAN_POINT('Origin',(3.86862915010152,9.,5.63137084989848));
#13001=CARTESIAN_POINT('Origin',(6.13137084989848,5.9,5.63137084989848));
#13002=CARTESIAN_POINT('',(5.96637084989848,6.,5.63137084989848));
#13003=CARTESIAN_POINT('Origin',(6.13137084989848,6.,5.63137084989848));
#13004=CARTESIAN_POINT('',(5.96637084989848,9.,5.63137084989848));
#13005=CARTESIAN_POINT('',(5.96637084989848,5.9,5.63137084989848));
#13006=CARTESIAN_POINT('Origin',(6.13137084989848,9.,5.63137084989848));
#13007=CARTESIAN_POINT('Origin',(6.13137084989848,5.9,3.36862915010152));
#13008=CARTESIAN_POINT('',(5.96637084989848,6.,3.36862915010152));
#13009=CARTESIAN_POINT('Origin',(6.13137084989848,6.,3.36862915010152));
#13010=CARTESIAN_POINT('',(5.96637084989848,9.,3.36862915010152));
#13011=CARTESIAN_POINT('',(5.96637084989848,5.9,3.36862915010152));
#13012=CARTESIAN_POINT('Origin',(6.13137084989848,9.,3.36862915010152));
#13013=CARTESIAN_POINT('Origin',(5.,5.9,4.5));
#13014=CARTESIAN_POINT('',(3.95,6.,4.5));
#13015=CARTESIAN_POINT('Origin',(5.,6.,4.5));
#13016=CARTESIAN_POINT('',(3.95,9.,4.5));
#13017=CARTESIAN_POINT('',(3.95,5.9,4.5));
#13018=CARTESIAN_POINT('Origin',(5.,9.,4.5));
#13019=CARTESIAN_POINT('Origin',(3.,6.,0.));
#13020=CARTESIAN_POINT('',(3.,6.,6.5));
#13021=CARTESIAN_POINT('',(3.,6.,0.));
#13022=CARTESIAN_POINT('',(3.,6.,6.5));
#13023=CARTESIAN_POINT('',(3.,9.,6.5));
#13024=CARTESIAN_POINT('',(3.,6.,6.5));
#13025=CARTESIAN_POINT('',(3.,9.,0.));
#13026=CARTESIAN_POINT('',(3.,9.,6.5));
#13027=CARTESIAN_POINT('',(3.,5.25,0.));
#13028=CARTESIAN_POINT('Origin',(7.,6.,6.5));
#13029=CARTESIAN_POINT('',(7.,6.,0.));
#13030=CARTESIAN_POINT('',(7.,6.,6.5));
#13031=CARTESIAN_POINT('',(7.,6.,0.));
#13032=CARTESIAN_POINT('',(7.,9.,0.));
#13033=CARTESIAN_POINT('',(7.,5.25,0.));
#13034=CARTESIAN_POINT('',(7.,9.,6.5));
#13035=CARTESIAN_POINT('',(7.,9.,0.));
#13036=CARTESIAN_POINT('',(7.,6.,6.5));
#13037=CARTESIAN_POINT('Origin',(3.,6.,6.5));
#13038=CARTESIAN_POINT('',(7.,6.,6.5));
#13039=CARTESIAN_POINT('',(7.,9.,6.5));
#13040=CARTESIAN_POINT('Origin',(5.,9.,3.25));
#13041=CARTESIAN_POINT('',(2.5,9.,0.));
#13042=CARTESIAN_POINT('Origin',(5.,6.,3.25));
#13043=CARTESIAN_POINT('',(2.5,6.,0.));
#13044=CARTESIAN_POINT('Origin',(-6.13137084989848,5.9,3.36862915010152));
#13045=CARTESIAN_POINT('',(-6.29637084989848,6.,3.36862915010152));
#13046=CARTESIAN_POINT('Origin',(-6.13137084989848,6.,3.36862915010152));
#13047=CARTESIAN_POINT('',(-6.29637084989848,9.,3.36862915010152));
#13048=CARTESIAN_POINT('',(-6.29637084989848,5.9,3.36862915010152));
#13049=CARTESIAN_POINT('Origin',(-6.13137084989848,9.,3.36862915010152));
#13050=CARTESIAN_POINT('Origin',(-6.13137084989848,5.9,5.63137084989848));
#13051=CARTESIAN_POINT('',(-6.29637084989848,6.,5.63137084989848));
#13052=CARTESIAN_POINT('Origin',(-6.13137084989848,6.,5.63137084989848));
#13053=CARTESIAN_POINT('',(-6.29637084989848,9.,5.63137084989848));
#13054=CARTESIAN_POINT('',(-6.29637084989848,5.9,5.63137084989848));
#13055=CARTESIAN_POINT('Origin',(-6.13137084989848,9.,5.63137084989848));
#13056=CARTESIAN_POINT('Origin',(-3.86862915010152,5.9,5.63137084989848));
#13057=CARTESIAN_POINT('',(-4.03362915010152,6.,5.63137084989848));
#13058=CARTESIAN_POINT('Origin',(-3.86862915010152,6.,5.63137084989848));
#13059=CARTESIAN_POINT('',(-4.03362915010152,9.,5.63137084989848));
#13060=CARTESIAN_POINT('',(-4.03362915010152,5.9,5.63137084989848));
#13061=CARTESIAN_POINT('Origin',(-3.86862915010152,9.,5.63137084989848));
#13062=CARTESIAN_POINT('Origin',(-3.86862915010152,5.9,3.36862915010152));
#13063=CARTESIAN_POINT('',(-4.03362915010152,6.,3.36862915010152));
#13064=CARTESIAN_POINT('Origin',(-3.86862915010152,6.,3.36862915010152));
#13065=CARTESIAN_POINT('',(-4.03362915010152,9.,3.36862915010152));
#13066=CARTESIAN_POINT('',(-4.03362915010152,5.9,3.36862915010152));
#13067=CARTESIAN_POINT('Origin',(-3.86862915010152,9.,3.36862915010152));
#13068=CARTESIAN_POINT('Origin',(-5.,5.9,4.5));
#13069=CARTESIAN_POINT('',(-6.05,6.,4.5));
#13070=CARTESIAN_POINT('Origin',(-5.,6.,4.5));
#13071=CARTESIAN_POINT('',(-6.05,9.,4.5));
#13072=CARTESIAN_POINT('',(-6.05,5.9,4.5));
#13073=CARTESIAN_POINT('Origin',(-5.,9.,4.5));
#13074=CARTESIAN_POINT('Origin',(-7.,6.,0.));
#13075=CARTESIAN_POINT('',(-7.,6.,6.5));
#13076=CARTESIAN_POINT('',(-7.,6.,0.));
#13077=CARTESIAN_POINT('',(-7.,6.,6.5));
#13078=CARTESIAN_POINT('',(-7.,9.,6.5));
#13079=CARTESIAN_POINT('',(-7.,6.,6.5));
#13080=CARTESIAN_POINT('',(-7.,9.,0.));
#13081=CARTESIAN_POINT('',(-7.,9.,6.5));
#13082=CARTESIAN_POINT('',(-7.,5.25,0.));
#13083=CARTESIAN_POINT('Origin',(-3.,6.,6.5));
#13084=CARTESIAN_POINT('',(-3.,6.,0.));
#13085=CARTESIAN_POINT('',(-3.,6.,6.5));
#13086=CARTESIAN_POINT('',(-3.,6.,0.));
#13087=CARTESIAN_POINT('',(-3.,9.,0.));
#13088=CARTESIAN_POINT('',(-3.,5.25,0.));
#13089=CARTESIAN_POINT('',(-3.,9.,6.5));
#13090=CARTESIAN_POINT('',(-3.,9.,0.));
#13091=CARTESIAN_POINT('',(-3.,6.,6.5));
#13092=CARTESIAN_POINT('Origin',(-7.,6.,6.5));
#13093=CARTESIAN_POINT('',(-3.,6.,6.5));
#13094=CARTESIAN_POINT('',(-3.,9.,6.5));
#13095=CARTESIAN_POINT('Origin',(-5.,9.,3.25));
#13096=CARTESIAN_POINT('',(-2.5,9.,0.));
#13097=CARTESIAN_POINT('Origin',(-5.,6.,3.25));
#13098=CARTESIAN_POINT('',(-2.5,6.,0.));
#13099=CARTESIAN_POINT('Origin',(7.5,13.5,-0.8));
#13100=CARTESIAN_POINT('',(7.5,13.5,-0.8));
#13101=CARTESIAN_POINT('',(-7.5,13.5,-0.8));
#13102=CARTESIAN_POINT('',(7.5,13.5,-0.8));
#13103=CARTESIAN_POINT('',(-7.5,13.5,0.));
#13104=CARTESIAN_POINT('',(-7.5,13.5,-0.8));
#13105=CARTESIAN_POINT('',(7.5,13.5,0.));
#13106=CARTESIAN_POINT('',(7.5,13.5,0.));
#13107=CARTESIAN_POINT('',(7.5,13.5,-0.8));
#13108=CARTESIAN_POINT('Origin',(7.5,-4.5,-0.8));
#13109=CARTESIAN_POINT('',(7.5,-4.5,-0.8));
#13110=CARTESIAN_POINT('',(7.5,-4.5,-0.8));
#13111=CARTESIAN_POINT('',(7.5,-4.5,0.));
#13112=CARTESIAN_POINT('',(7.5,-4.5,0.));
#13113=CARTESIAN_POINT('',(7.5,-4.5,-0.8));
#13114=CARTESIAN_POINT('Origin',(-7.5,-4.5,-0.8));
#13115=CARTESIAN_POINT('',(-7.5,-4.5,-0.8));
#13116=CARTESIAN_POINT('',(-7.5,-4.5,-0.8));
#13117=CARTESIAN_POINT('',(-7.5,-4.5,0.));
#13118=CARTESIAN_POINT('',(-7.5,-4.5,0.));
#13119=CARTESIAN_POINT('',(-7.5,-4.5,-0.8));
#13120=CARTESIAN_POINT('Origin',(-7.5,13.5,-0.8));
#13121=CARTESIAN_POINT('',(-7.5,13.5,-0.8));
#13122=CARTESIAN_POINT('',(-7.5,13.5,0.));
#13123=CARTESIAN_POINT('Origin',(0.,4.5,0.));
#13124=CARTESIAN_POINT('Origin',(0.,4.5,-0.8));
#14319=UNCERTAINTY_MEASURE_WITH_UNIT(LENGTH_MEASURE(0.001),#14393,
'DISTANCE_ACCURACY_VALUE',
'Maximum model space distance between geometric entities at asserted c
onnectivities');
#14344=UNCERTAINTY_MEASURE_WITH_UNIT(LENGTH_MEASURE(0.001),#14393,
'DISTANCE_ACCURACY_VALUE',
'Maximum model space distance between geometric entities at asserted c
onnectivities');
#14367=(
GEOMETRIC_REPRESENTATION_CONTEXT(3)
GLOBAL_UNCERTAINTY_ASSIGNED_CONTEXT((#14319))
GLOBAL_UNIT_ASSIGNED_CONTEXT((#14393,#14395,#14396))
REPRESENTATION_CONTEXT('','3D')
);
#14392=(
GEOMETRIC_REPRESENTATION_CONTEXT(3)
GLOBAL_UNCERTAINTY_ASSIGNED_CONTEXT((#14344))
GLOBAL_UNIT_ASSIGNED_CONTEXT((#14393,#14395,#14396))
REPRESENTATION_CONTEXT('','3D')
);
#14393=(
LENGTH_UNIT()
NAMED_UNIT(*)
SI_UNIT(.CENTI.,.METRE.)
);
#14395=(
NAMED_UNIT(*)
PLANE_ANGLE_UNIT()
SI_UNIT($,.RADIAN.)
);
#14396=(
NAMED_UNIT(*)
SI_UNIT($,.STERADIAN.)
SOLID_ANGLE_UNIT()
);
#14419=SHAPE_DEFINITION_REPRESENTATION(#14468,#14605);
#14468=PRODUCT_DEFINITION_SHAPE('',$,#14653);
#14605=SHAPE_REPRESENTATION('',(#8825),#14367);
#14630=PRODUCT_DEFINITION_CONTEXT('part definition',#14773,'design');
#14653=PRODUCT_DEFINITION('Cylinder and guide mounting frame',
'Cylinder and guide mounting frame',#14700,#14630);
#14700=PRODUCT_DEFINITION_FORMATION('',$,#14797);
#14773=APPLICATION_CONTEXT(
'Core Data for Automotive Mechanical Design Process');
#14774=PRODUCT_CONTEXT('part definition',#14773,'mechanical');
#14797=PRODUCT('Cylinder and guide mounting frame',
'Cylinder and guide mounting frame','Cylinder and guide mounting frame',
(#14774));
#14864=COLOUR_RGB('Dark Blue',0.08,0.2,0.34);
#14865=FILL_AREA_STYLE_COLOUR('',#14864);
#14866=FILL_AREA_STYLE('',(#14865));
#14867=SURFACE_STYLE_FILL_AREA(#14866);
#14868=SURFACE_SIDE_STYLE('',(#14867));
#14869=SURFACE_STYLE_USAGE(.BOTH.,#14868);
#14870=PRESENTATION_STYLE_ASSIGNMENT((#14869));
ENDSEC;
END-ISO-10303-21;
